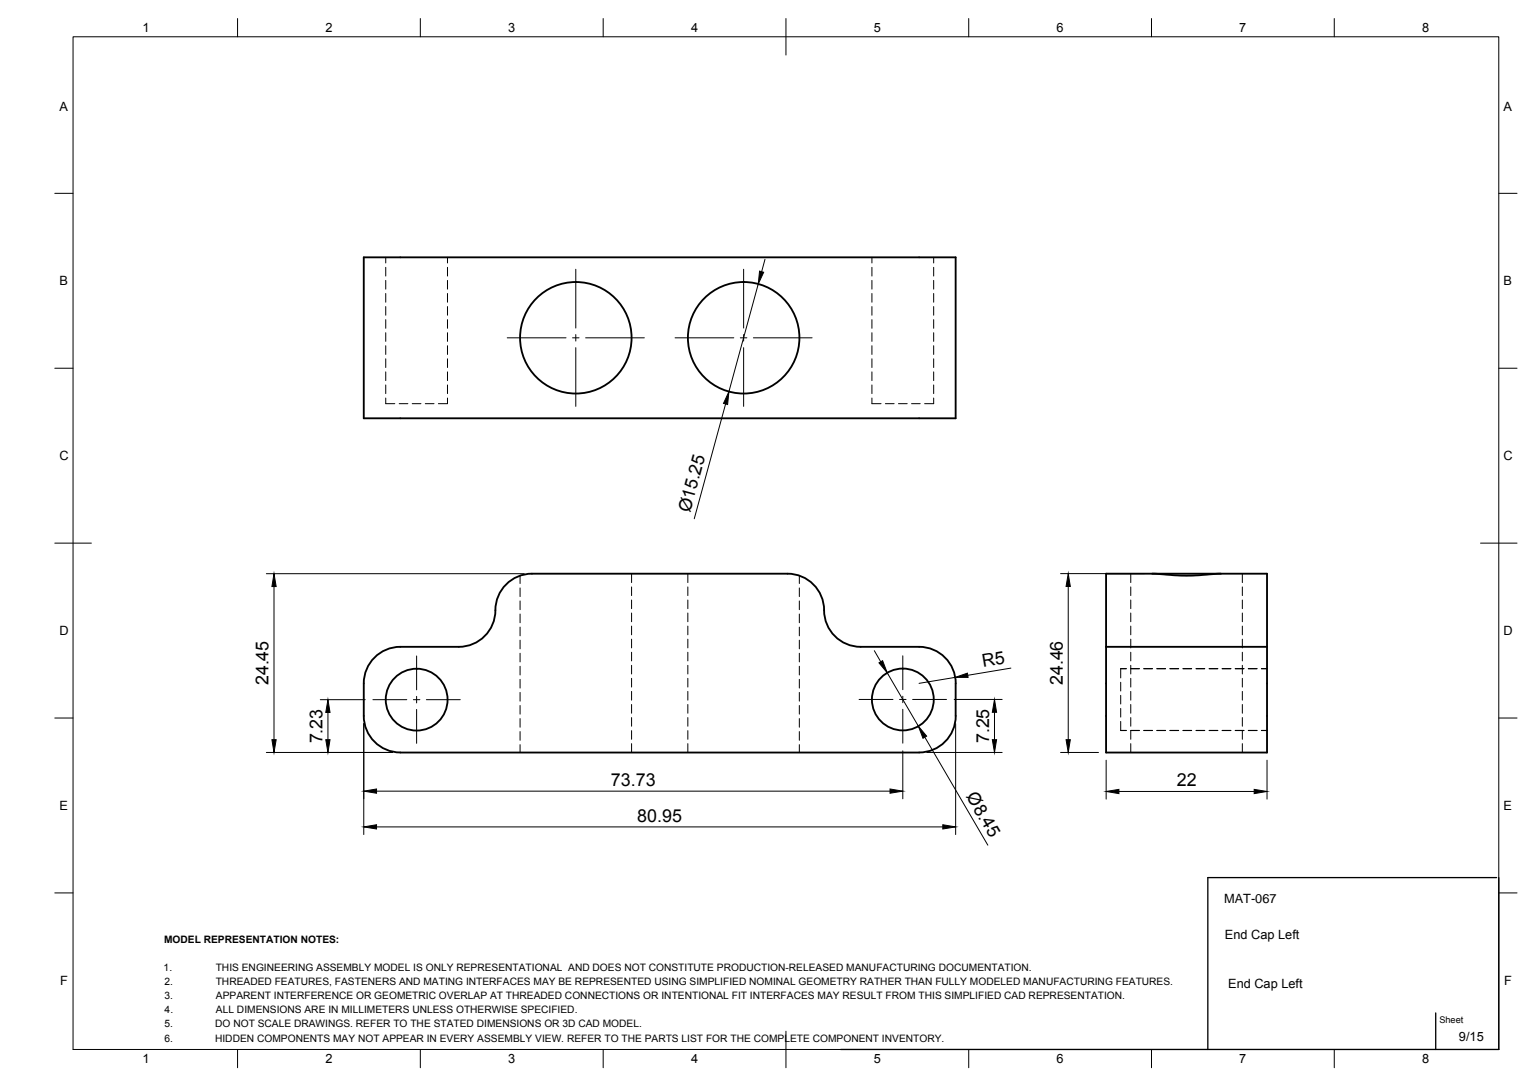
ISO-10303-21;
HEADER;
/* Generated by software containing ST-Developer
 * from STEP Tools, Inc. (www.steptools.com) 
 */

FILE_DESCRIPTION(
/* description */ ('CAx-IF Rec.Pracs.---Representation and Presentation of Product Manufa
cturing Information (PMI)---4.0---2014-10-13'),
/* implementation_level */ '2;1');

FILE_NAME(
/* name */ 'End Cap Left.step',
/* time_stamp */ '2026-10-24T16:02:03-07:00',
/* author */ (''),
/* organization */ (''),
/* preprocessor_version */ 'ST-DEVELOPER v20.2',
/* originating_system */ 'Autodesk Translation Framework v15.17.0.0',
/* authorisation */ '');

FILE_SCHEMA (('AP242_MANAGED_MODEL_BASED_3D_ENGINEERING_MIM_LF { 1 0 10303 442 2 1 4 }'));
ENDSEC;

DATA;
#10=MECHANICAL_DESIGN_GEOMETRIC_PRESENTATION_REPRESENTATION('',(#354),#6348);
#332=SHAPE_REPRESENTATION_RELATIONSHIP('SRR','None',#6483,#343);
#343=ADVANCED_BREP_SHAPE_REPRESENTATION('',(#365),#6331);
#354=STYLED_ITEM('',(#6604),#365);
#365=MANIFOLD_SOLID_BREP('Body1',#3393);
#382=B_SPLINE_CURVE_WITH_KNOTS('',3,(#5983,#5984,#5985,#5986,#5987,#5988),
 .UNSPECIFIED.,.F.,.F.,(4,2,4),(3.46797062946804,3.66737221611079,3.95578831781598),
 .UNSPECIFIED.);
#383=B_SPLINE_CURVE_WITH_KNOTS('',3,(#5989,#5990,#5991,#5992,#5993,#5994),
 .UNSPECIFIED.,.F.,.F.,(4,2,4),(3.95578831781598,4.24420441952117,4.44360600616391),
 .UNSPECIFIED.);
#384=B_SPLINE_CURVE_WITH_KNOTS('',3,(#5997,#5998,#5999,#6000,#6001,#6002,
#6003,#6004,#6005,#6006),.UNSPECIFIED.,.F.,.F.,(4,2,2,2,4),(-4.44360600616391,
-4.24420441952117,-3.95578831781597,-3.66737221611078,-3.46797062946804),
 .UNSPECIFIED.);
#433=CYLINDRICAL_SURFACE('',#3738,0.004225);
#434=CYLINDRICAL_SURFACE('',#3742,0.004225);
#435=CYLINDRICAL_SURFACE('',#3765,0.005);
#436=CYLINDRICAL_SURFACE('',#3766,0.005);
#437=CYLINDRICAL_SURFACE('',#3767,0.005);
#438=CYLINDRICAL_SURFACE('',#3768,0.005);
#439=CYLINDRICAL_SURFACE('',#3773,0.007625);
#440=CYLINDRICAL_SURFACE('',#3774,0.007625);
#441=CYLINDRICAL_SURFACE('',#3775,0.005);
#442=CYLINDRICAL_SURFACE('',#3776,0.005);
#443=CYLINDRICAL_SURFACE('',#3777,0.005);
#444=CYLINDRICAL_SURFACE('',#3778,0.005);
#484=FACE_BOUND('',#986,.T.);
#485=FACE_BOUND('',#987,.T.);
#486=FACE_BOUND('',#993,.T.);
#487=FACE_BOUND('',#994,.T.);
#611=CIRCLE('',#3735,0.007625);
#612=CIRCLE('',#3736,0.007625);
#613=CIRCLE('',#3739,0.004225);
#614=CIRCLE('',#3740,0.004225);
#615=CIRCLE('',#3743,0.004225);
#616=CIRCLE('',#3744,0.004225);
#617=CIRCLE('',#3746,0.005);
#618=CIRCLE('',#3747,0.005);
#619=CIRCLE('',#3748,0.005);
#620=CIRCLE('',#3749,0.005);
#621=CIRCLE('',#3750,0.005);
#622=CIRCLE('',#3751,0.005);
#623=CIRCLE('',#3752,0.005);
#624=CIRCLE('',#3753,0.005);
#625=CIRCLE('',#3757,0.005);
#626=CIRCLE('',#3758,0.005);
#627=CIRCLE('',#3759,0.005);
#628=CIRCLE('',#3760,0.005);
#629=CIRCLE('',#3761,0.005);
#630=CIRCLE('',#3762,0.005);
#631=CIRCLE('',#3763,0.005);
#632=CIRCLE('',#3764,0.005);
#633=CIRCLE('',#3770,0.007625);
#634=CIRCLE('',#3771,0.007625);
#635=CIRCLE('',#3772,0.007625);
#792=FACE_OUTER_BOUND('',#983,.T.);
#793=FACE_OUTER_BOUND('',#984,.T.);
#794=FACE_OUTER_BOUND('',#985,.T.);
#795=FACE_OUTER_BOUND('',#988,.T.);
#796=FACE_OUTER_BOUND('',#989,.T.);
#797=FACE_OUTER_BOUND('',#990,.T.);
#798=FACE_OUTER_BOUND('',#991,.T.);
#799=FACE_OUTER_BOUND('',#992,.T.);
#800=FACE_OUTER_BOUND('',#995,.T.);
#801=FACE_OUTER_BOUND('',#996,.T.);
#802=FACE_OUTER_BOUND('',#997,.T.);
#803=FACE_OUTER_BOUND('',#998,.T.);
#804=FACE_OUTER_BOUND('',#999,.T.);
#805=FACE_OUTER_BOUND('',#1000,.T.);
#806=FACE_OUTER_BOUND('',#1001,.T.);
#807=FACE_OUTER_BOUND('',#1002,.T.);
#808=FACE_OUTER_BOUND('',#1003,.T.);
#809=FACE_OUTER_BOUND('',#1004,.T.);
#810=FACE_OUTER_BOUND('',#1005,.T.);
#811=FACE_OUTER_BOUND('',#1006,.T.);
#812=FACE_OUTER_BOUND('',#1007,.T.);
#813=FACE_OUTER_BOUND('',#1008,.T.);
#983=EDGE_LOOP('',(#2843,#2844,#2845,#2846));
#984=EDGE_LOOP('',(#2847,#2848,#2849,#2850));
#985=EDGE_LOOP('',(#2851,#2852,#2853,#2854));
#986=EDGE_LOOP('',(#2855));
#987=EDGE_LOOP('',(#2856));
#988=EDGE_LOOP('',(#2857,#2858,#2859,#2860));
#989=EDGE_LOOP('',(#2861,#2862,#2863,#2864));
#990=EDGE_LOOP('',(#2865,#2866,#2867,#2868));
#991=EDGE_LOOP('',(#2869,#2870,#2871,#2872));
#992=EDGE_LOOP('',(#2873,#2874,#2875,#2876,#2877,#2878,#2879,#2880,#2881,
#2882,#2883,#2884,#2885,#2886));
#993=EDGE_LOOP('',(#2887));
#994=EDGE_LOOP('',(#2888));
#995=EDGE_LOOP('',(#2889));
#996=EDGE_LOOP('',(#2890));
#997=EDGE_LOOP('',(#2891,#2892,#2893,#2894,#2895,#2896,#2897,#2898,#2899,
#2900,#2901,#2902,#2903,#2904));
#998=EDGE_LOOP('',(#2905,#2906,#2907,#2908));
#999=EDGE_LOOP('',(#2909,#2910,#2911,#2912));
#1000=EDGE_LOOP('',(#2913,#2914,#2915,#2916));
#1001=EDGE_LOOP('',(#2917,#2918,#2919,#2920));
#1002=EDGE_LOOP('',(#2921,#2922,#2923,#2924,#2925,#2926,#2927,#2928,#2929));
#1003=EDGE_LOOP('',(#2930,#2931,#2932,#2933,#2934,#2935));
#1004=EDGE_LOOP('',(#2936,#2937,#2938,#2939,#2940,#2941));
#1005=EDGE_LOOP('',(#2942,#2943,#2944,#2945,#2946,#2947));
#1006=EDGE_LOOP('',(#2948,#2949,#2950,#2951));
#1007=EDGE_LOOP('',(#2952,#2953,#2954,#2955,#2956,#2957,#2958));
#1008=EDGE_LOOP('',(#2959,#2960,#2961,#2962));
#1250=LINE('',#5875,#1483);
#1251=LINE('',#5877,#1484);
#1252=LINE('',#5879,#1485);
#1253=LINE('',#5880,#1486);
#1254=LINE('',#5884,#1487);
#1255=LINE('',#5886,#1488);
#1256=LINE('',#5888,#1489);
#1257=LINE('',#5889,#1490);
#1258=LINE('',#5893,#1491);
#1259=LINE('',#5895,#1492);
#1260=LINE('',#5897,#1493);
#1261=LINE('',#5898,#1494);
#1262=LINE('',#5906,#1495);
#1263=LINE('',#5908,#1496);
#1264=LINE('',#5910,#1497);
#1265=LINE('',#5911,#1498);
#1266=LINE('',#5916,#1499);
#1267=LINE('',#5921,#1500);
#1268=LINE('',#5923,#1501);
#1269=LINE('',#5925,#1502);
#1270=LINE('',#5926,#1503);
#1271=LINE('',#5931,#1504);
#1272=LINE('',#5936,#1505);
#1273=LINE('',#5955,#1506);
#1274=LINE('',#5969,#1507);
#1275=LINE('',#5974,#1508);
#1276=LINE('',#5976,#1509);
#1277=LINE('',#5979,#1510);
#1278=LINE('',#5982,#1511);
#1279=LINE('',#5996,#1512);
#1280=LINE('',#6008,#1513);
#1281=LINE('',#6011,#1514);
#1483=VECTOR('',#4576,1.);
#1484=VECTOR('',#4577,1.);
#1485=VECTOR('',#4578,1.);
#1486=VECTOR('',#4579,1.);
#1487=VECTOR('',#4582,1.);
#1488=VECTOR('',#4583,1.);
#1489=VECTOR('',#4584,1.);
#1490=VECTOR('',#4585,1.);
#1491=VECTOR('',#4588,1.);
#1492=VECTOR('',#4589,1.);
#1493=VECTOR('',#4590,1.);
#1494=VECTOR('',#4591,1.);
#1495=VECTOR('',#4598,1.);
#1496=VECTOR('',#4599,1.);
#1497=VECTOR('',#4600,1.);
#1498=VECTOR('',#4601,1.);
#1499=VECTOR('',#4606,0.004225);
#1500=VECTOR('',#4611,1.);
#1501=VECTOR('',#4612,1.);
#1502=VECTOR('',#4613,1.);
#1503=VECTOR('',#4614,1.);
#1504=VECTOR('',#4619,0.004225);
#1505=VECTOR('',#4624,1.);
#1506=VECTOR('',#4651,1.);
#1507=VECTOR('',#4674,1.);
#1508=VECTOR('',#4679,1.);
#1509=VECTOR('',#4680,1.);
#1510=VECTOR('',#4683,1.);
#1511=VECTOR('',#4686,0.007625);
#1512=VECTOR('',#4689,0.007625);
#1513=VECTOR('',#4692,1.);
#1514=VECTOR('',#4697,1.);
#1736=VERTEX_POINT('',#5873);
#1737=VERTEX_POINT('',#5874);
#1738=VERTEX_POINT('',#5876);
#1739=VERTEX_POINT('',#5878);
#1740=VERTEX_POINT('',#5882);
#1741=VERTEX_POINT('',#5883);
#1742=VERTEX_POINT('',#5885);
#1743=VERTEX_POINT('',#5887);
#1744=VERTEX_POINT('',#5891);
#1745=VERTEX_POINT('',#5892);
#1746=VERTEX_POINT('',#5894);
#1747=VERTEX_POINT('',#5896);
#1748=VERTEX_POINT('',#5899);
#1749=VERTEX_POINT('',#5901);
#1750=VERTEX_POINT('',#5904);
#1751=VERTEX_POINT('',#5905);
#1752=VERTEX_POINT('',#5907);
#1753=VERTEX_POINT('',#5909);
#1754=VERTEX_POINT('',#5913);
#1755=VERTEX_POINT('',#5915);
#1756=VERTEX_POINT('',#5919);
#1757=VERTEX_POINT('',#5920);
#1758=VERTEX_POINT('',#5922);
#1759=VERTEX_POINT('',#5924);
#1760=VERTEX_POINT('',#5928);
#1761=VERTEX_POINT('',#5930);
#1762=VERTEX_POINT('',#5934);
#1763=VERTEX_POINT('',#5935);
#1764=VERTEX_POINT('',#5937);
#1765=VERTEX_POINT('',#5944);
#1766=VERTEX_POINT('',#5950);
#1767=VERTEX_POINT('',#5952);
#1768=VERTEX_POINT('',#5954);
#1769=VERTEX_POINT('',#5956);
#1770=VERTEX_POINT('',#5968);
#1771=VERTEX_POINT('',#5970);
#1772=VERTEX_POINT('',#5972);
#1773=VERTEX_POINT('',#5975);
#1774=VERTEX_POINT('',#5977);
#1775=VERTEX_POINT('',#5981);
#2120=EDGE_CURVE('',#1736,#1737,#1250,.T.);
#2121=EDGE_CURVE('',#1736,#1738,#1251,.F.);
#2122=EDGE_CURVE('',#1738,#1739,#1252,.T.);
#2123=EDGE_CURVE('',#1739,#1737,#1253,.T.);
#2124=EDGE_CURVE('',#1740,#1741,#1254,.T.);
#2125=EDGE_CURVE('',#1741,#1742,#1255,.T.);
#2126=EDGE_CURVE('',#1743,#1742,#1256,.T.);
#2127=EDGE_CURVE('',#1743,#1740,#1257,.F.);
#2128=EDGE_CURVE('',#1744,#1745,#1258,.T.);
#2129=EDGE_CURVE('',#1744,#1746,#1259,.T.);
#2130=EDGE_CURVE('',#1746,#1747,#1260,.T.);
#2131=EDGE_CURVE('',#1747,#1745,#1261,.F.);
#2132=EDGE_CURVE('',#1748,#1748,#611,.T.);
#2133=EDGE_CURVE('',#1749,#1749,#612,.T.);
#2134=EDGE_CURVE('',#1750,#1751,#1262,.T.);
#2135=EDGE_CURVE('',#1750,#1752,#1263,.T.);
#2136=EDGE_CURVE('',#1752,#1753,#1264,.T.);
#2137=EDGE_CURVE('',#1753,#1751,#1265,.F.);
#2138=EDGE_CURVE('',#1754,#1754,#613,.T.);
#2139=EDGE_CURVE('',#1754,#1755,#1266,.T.);
#2140=EDGE_CURVE('',#1755,#1755,#614,.T.);
#2141=EDGE_CURVE('',#1756,#1757,#1267,.T.);
#2142=EDGE_CURVE('',#1757,#1758,#1268,.T.);
#2143=EDGE_CURVE('',#1759,#1758,#1269,.T.);
#2144=EDGE_CURVE('',#1759,#1756,#1270,.F.);
#2145=EDGE_CURVE('',#1760,#1760,#615,.T.);
#2146=EDGE_CURVE('',#1760,#1761,#1271,.T.);
#2147=EDGE_CURVE('',#1761,#1761,#616,.T.);
#2148=EDGE_CURVE('',#1762,#1763,#1272,.T.);
#2149=EDGE_CURVE('',#1763,#1764,#617,.F.);
#2150=EDGE_CURVE('',#1764,#1736,#618,.T.);
#2151=EDGE_CURVE('',#1737,#1753,#619,.F.);
#2152=EDGE_CURVE('',#1752,#1747,#620,.F.);
#2153=EDGE_CURVE('',#1746,#1743,#621,.F.);
#2154=EDGE_CURVE('',#1742,#1759,#622,.F.);
#2155=EDGE_CURVE('',#1758,#1765,#623,.T.);
#2156=EDGE_CURVE('',#1765,#1762,#624,.F.);
#2157=EDGE_CURVE('',#1738,#1766,#625,.F.);
#2158=EDGE_CURVE('',#1766,#1767,#626,.T.);
#2159=EDGE_CURVE('',#1768,#1767,#1273,.T.);
#2160=EDGE_CURVE('',#1768,#1769,#627,.T.);
#2161=EDGE_CURVE('',#1769,#1757,#628,.F.);
#2162=EDGE_CURVE('',#1756,#1741,#629,.T.);
#2163=EDGE_CURVE('',#1740,#1744,#630,.T.);
#2164=EDGE_CURVE('',#1745,#1750,#631,.T.);
#2165=EDGE_CURVE('',#1751,#1739,#632,.T.);
#2166=EDGE_CURVE('',#1767,#1770,#1274,.T.);
#2167=EDGE_CURVE('',#1771,#1770,#633,.T.);
#2168=EDGE_CURVE('',#1772,#1771,#634,.T.);
#2169=EDGE_CURVE('',#1772,#1763,#1275,.T.);
#2170=EDGE_CURVE('',#1762,#1773,#1276,.F.);
#2171=EDGE_CURVE('',#1774,#1773,#635,.T.);
#2172=EDGE_CURVE('',#1774,#1768,#1277,.F.);
#2173=EDGE_CURVE('',#1749,#1775,#1278,.T.);
#2174=EDGE_CURVE('',#1775,#1774,#382,.F.);
#2175=EDGE_CURVE('',#1773,#1775,#383,.F.);
#2176=EDGE_CURVE('',#1748,#1771,#1279,.T.);
#2177=EDGE_CURVE('',#1770,#1772,#384,.T.);
#2178=EDGE_CURVE('',#1764,#1766,#1280,.F.);
#2179=EDGE_CURVE('',#1769,#1765,#1281,.T.);
#2843=ORIENTED_EDGE('',*,*,#2120,.F.);
#2844=ORIENTED_EDGE('',*,*,#2121,.T.);
#2845=ORIENTED_EDGE('',*,*,#2122,.T.);
#2846=ORIENTED_EDGE('',*,*,#2123,.T.);
#2847=ORIENTED_EDGE('',*,*,#2124,.T.);
#2848=ORIENTED_EDGE('',*,*,#2125,.T.);
#2849=ORIENTED_EDGE('',*,*,#2126,.F.);
#2850=ORIENTED_EDGE('',*,*,#2127,.T.);
#2851=ORIENTED_EDGE('',*,*,#2128,.F.);
#2852=ORIENTED_EDGE('',*,*,#2129,.T.);
#2853=ORIENTED_EDGE('',*,*,#2130,.T.);
#2854=ORIENTED_EDGE('',*,*,#2131,.T.);
#2855=ORIENTED_EDGE('',*,*,#2132,.T.);
#2856=ORIENTED_EDGE('',*,*,#2133,.T.);
#2857=ORIENTED_EDGE('',*,*,#2134,.F.);
#2858=ORIENTED_EDGE('',*,*,#2135,.T.);
#2859=ORIENTED_EDGE('',*,*,#2136,.T.);
#2860=ORIENTED_EDGE('',*,*,#2137,.T.);
#2861=ORIENTED_EDGE('',*,*,#2138,.T.);
#2862=ORIENTED_EDGE('',*,*,#2139,.T.);
#2863=ORIENTED_EDGE('',*,*,#2140,.F.);
#2864=ORIENTED_EDGE('',*,*,#2139,.F.);
#2865=ORIENTED_EDGE('',*,*,#2141,.T.);
#2866=ORIENTED_EDGE('',*,*,#2142,.T.);
#2867=ORIENTED_EDGE('',*,*,#2143,.F.);
#2868=ORIENTED_EDGE('',*,*,#2144,.T.);
#2869=ORIENTED_EDGE('',*,*,#2145,.T.);
#2870=ORIENTED_EDGE('',*,*,#2146,.T.);
#2871=ORIENTED_EDGE('',*,*,#2147,.F.);
#2872=ORIENTED_EDGE('',*,*,#2146,.F.);
#2873=ORIENTED_EDGE('',*,*,#2148,.T.);
#2874=ORIENTED_EDGE('',*,*,#2149,.T.);
#2875=ORIENTED_EDGE('',*,*,#2150,.T.);
#2876=ORIENTED_EDGE('',*,*,#2120,.T.);
#2877=ORIENTED_EDGE('',*,*,#2151,.T.);
#2878=ORIENTED_EDGE('',*,*,#2136,.F.);
#2879=ORIENTED_EDGE('',*,*,#2152,.T.);
#2880=ORIENTED_EDGE('',*,*,#2130,.F.);
#2881=ORIENTED_EDGE('',*,*,#2153,.T.);
#2882=ORIENTED_EDGE('',*,*,#2126,.T.);
#2883=ORIENTED_EDGE('',*,*,#2154,.T.);
#2884=ORIENTED_EDGE('',*,*,#2143,.T.);
#2885=ORIENTED_EDGE('',*,*,#2155,.T.);
#2886=ORIENTED_EDGE('',*,*,#2156,.T.);
#2887=ORIENTED_EDGE('',*,*,#2140,.T.);
#2888=ORIENTED_EDGE('',*,*,#2147,.T.);
#2889=ORIENTED_EDGE('',*,*,#2145,.F.);
#2890=ORIENTED_EDGE('',*,*,#2138,.F.);
#2891=ORIENTED_EDGE('',*,*,#2122,.F.);
#2892=ORIENTED_EDGE('',*,*,#2157,.T.);
#2893=ORIENTED_EDGE('',*,*,#2158,.T.);
#2894=ORIENTED_EDGE('',*,*,#2159,.F.);
#2895=ORIENTED_EDGE('',*,*,#2160,.T.);
#2896=ORIENTED_EDGE('',*,*,#2161,.T.);
#2897=ORIENTED_EDGE('',*,*,#2141,.F.);
#2898=ORIENTED_EDGE('',*,*,#2162,.T.);
#2899=ORIENTED_EDGE('',*,*,#2124,.F.);
#2900=ORIENTED_EDGE('',*,*,#2163,.T.);
#2901=ORIENTED_EDGE('',*,*,#2128,.T.);
#2902=ORIENTED_EDGE('',*,*,#2164,.T.);
#2903=ORIENTED_EDGE('',*,*,#2134,.T.);
#2904=ORIENTED_EDGE('',*,*,#2165,.T.);
#2905=ORIENTED_EDGE('',*,*,#2162,.F.);
#2906=ORIENTED_EDGE('',*,*,#2144,.F.);
#2907=ORIENTED_EDGE('',*,*,#2154,.F.);
#2908=ORIENTED_EDGE('',*,*,#2125,.F.);
#2909=ORIENTED_EDGE('',*,*,#2163,.F.);
#2910=ORIENTED_EDGE('',*,*,#2127,.F.);
#2911=ORIENTED_EDGE('',*,*,#2153,.F.);
#2912=ORIENTED_EDGE('',*,*,#2129,.F.);
#2913=ORIENTED_EDGE('',*,*,#2164,.F.);
#2914=ORIENTED_EDGE('',*,*,#2131,.F.);
#2915=ORIENTED_EDGE('',*,*,#2152,.F.);
#2916=ORIENTED_EDGE('',*,*,#2135,.F.);
#2917=ORIENTED_EDGE('',*,*,#2165,.F.);
#2918=ORIENTED_EDGE('',*,*,#2137,.F.);
#2919=ORIENTED_EDGE('',*,*,#2151,.F.);
#2920=ORIENTED_EDGE('',*,*,#2123,.F.);
#2921=ORIENTED_EDGE('',*,*,#2159,.T.);
#2922=ORIENTED_EDGE('',*,*,#2166,.T.);
#2923=ORIENTED_EDGE('',*,*,#2167,.F.);
#2924=ORIENTED_EDGE('',*,*,#2168,.F.);
#2925=ORIENTED_EDGE('',*,*,#2169,.T.);
#2926=ORIENTED_EDGE('',*,*,#2148,.F.);
#2927=ORIENTED_EDGE('',*,*,#2170,.T.);
#2928=ORIENTED_EDGE('',*,*,#2171,.F.);
#2929=ORIENTED_EDGE('',*,*,#2172,.T.);
#2930=ORIENTED_EDGE('',*,*,#2133,.F.);
#2931=ORIENTED_EDGE('',*,*,#2173,.T.);
#2932=ORIENTED_EDGE('',*,*,#2174,.T.);
#2933=ORIENTED_EDGE('',*,*,#2171,.T.);
#2934=ORIENTED_EDGE('',*,*,#2175,.T.);
#2935=ORIENTED_EDGE('',*,*,#2173,.F.);
#2936=ORIENTED_EDGE('',*,*,#2132,.F.);
#2937=ORIENTED_EDGE('',*,*,#2176,.T.);
#2938=ORIENTED_EDGE('',*,*,#2167,.T.);
#2939=ORIENTED_EDGE('',*,*,#2177,.T.);
#2940=ORIENTED_EDGE('',*,*,#2168,.T.);
#2941=ORIENTED_EDGE('',*,*,#2176,.F.);
#2942=ORIENTED_EDGE('',*,*,#2166,.F.);
#2943=ORIENTED_EDGE('',*,*,#2158,.F.);
#2944=ORIENTED_EDGE('',*,*,#2178,.F.);
#2945=ORIENTED_EDGE('',*,*,#2149,.F.);
#2946=ORIENTED_EDGE('',*,*,#2169,.F.);
#2947=ORIENTED_EDGE('',*,*,#2177,.F.);
#2948=ORIENTED_EDGE('',*,*,#2157,.F.);
#2949=ORIENTED_EDGE('',*,*,#2121,.F.);
#2950=ORIENTED_EDGE('',*,*,#2150,.F.);
#2951=ORIENTED_EDGE('',*,*,#2178,.T.);
#2952=ORIENTED_EDGE('',*,*,#2179,.F.);
#2953=ORIENTED_EDGE('',*,*,#2160,.F.);
#2954=ORIENTED_EDGE('',*,*,#2172,.F.);
#2955=ORIENTED_EDGE('',*,*,#2174,.F.);
#2956=ORIENTED_EDGE('',*,*,#2175,.F.);
#2957=ORIENTED_EDGE('',*,*,#2170,.F.);
#2958=ORIENTED_EDGE('',*,*,#2156,.F.);
#2959=ORIENTED_EDGE('',*,*,#2161,.F.);
#2960=ORIENTED_EDGE('',*,*,#2179,.T.);
#2961=ORIENTED_EDGE('',*,*,#2155,.F.);
#2962=ORIENTED_EDGE('',*,*,#2142,.F.);
#3187=PLANE('',#3732);
#3188=PLANE('',#3733);
#3189=PLANE('',#3734);
#3190=PLANE('',#3737);
#3191=PLANE('',#3741);
#3192=PLANE('',#3745);
#3193=PLANE('',#3754);
#3194=PLANE('',#3755);
#3195=PLANE('',#3756);
#3196=PLANE('',#3769);
#3315=ADVANCED_FACE('',(#792),#3187,.T.);
#3316=ADVANCED_FACE('',(#793),#3188,.T.);
#3317=ADVANCED_FACE('',(#794,#484,#485),#3189,.F.);
#3318=ADVANCED_FACE('',(#795),#3190,.F.);
#3319=ADVANCED_FACE('',(#796),#433,.F.);
#3320=ADVANCED_FACE('',(#797),#3191,.T.);
#3321=ADVANCED_FACE('',(#798),#434,.F.);
#3322=ADVANCED_FACE('',(#799,#486,#487),#3192,.F.);
#3323=ADVANCED_FACE('',(#800),#3193,.F.);
#3324=ADVANCED_FACE('',(#801),#3194,.F.);
#3325=ADVANCED_FACE('',(#802),#3195,.T.);
#3326=ADVANCED_FACE('',(#803),#435,.T.);
#3327=ADVANCED_FACE('',(#804),#436,.T.);
#3328=ADVANCED_FACE('',(#805),#437,.T.);
#3329=ADVANCED_FACE('',(#806),#438,.T.);
#3330=ADVANCED_FACE('',(#807),#3196,.T.);
#3331=ADVANCED_FACE('',(#808),#439,.F.);
#3332=ADVANCED_FACE('',(#809),#440,.F.);
#3333=ADVANCED_FACE('',(#810),#441,.T.);
#3334=ADVANCED_FACE('',(#811),#442,.F.);
#3335=ADVANCED_FACE('',(#812),#443,.T.);
#3336=ADVANCED_FACE('',(#813),#444,.F.);
#3393=CLOSED_SHELL('',(#3315,#3316,#3317,#3318,#3319,#3320,#3321,#3322,
#3323,#3324,#3325,#3326,#3327,#3328,#3329,#3330,#3331,#3332,#3333,#3334,
#3335,#3336));
#3731=AXIS2_PLACEMENT_3D('',#5871,#4572,#4573);
#3732=AXIS2_PLACEMENT_3D('',#5872,#4574,#4575);
#3733=AXIS2_PLACEMENT_3D('',#5881,#4580,#4581);
#3734=AXIS2_PLACEMENT_3D('',#5890,#4586,#4587);
#3735=AXIS2_PLACEMENT_3D('',#5900,#4592,#4593);
#3736=AXIS2_PLACEMENT_3D('',#5902,#4594,#4595);
#3737=AXIS2_PLACEMENT_3D('',#5903,#4596,#4597);
#3738=AXIS2_PLACEMENT_3D('',#5912,#4602,#4603);
#3739=AXIS2_PLACEMENT_3D('',#5914,#4604,#4605);
#3740=AXIS2_PLACEMENT_3D('',#5917,#4607,#4608);
#3741=AXIS2_PLACEMENT_3D('',#5918,#4609,#4610);
#3742=AXIS2_PLACEMENT_3D('',#5927,#4615,#4616);
#3743=AXIS2_PLACEMENT_3D('',#5929,#4617,#4618);
#3744=AXIS2_PLACEMENT_3D('',#5932,#4620,#4621);
#3745=AXIS2_PLACEMENT_3D('',#5933,#4622,#4623);
#3746=AXIS2_PLACEMENT_3D('',#5938,#4625,#4626);
#3747=AXIS2_PLACEMENT_3D('',#5939,#4627,#4628);
#3748=AXIS2_PLACEMENT_3D('',#5940,#4629,#4630);
#3749=AXIS2_PLACEMENT_3D('',#5941,#4631,#4632);
#3750=AXIS2_PLACEMENT_3D('',#5942,#4633,#4634);
#3751=AXIS2_PLACEMENT_3D('',#5943,#4635,#4636);
#3752=AXIS2_PLACEMENT_3D('',#5945,#4637,#4638);
#3753=AXIS2_PLACEMENT_3D('',#5946,#4639,#4640);
#3754=AXIS2_PLACEMENT_3D('',#5947,#4641,#4642);
#3755=AXIS2_PLACEMENT_3D('',#5948,#4643,#4644);
#3756=AXIS2_PLACEMENT_3D('',#5949,#4645,#4646);
#3757=AXIS2_PLACEMENT_3D('',#5951,#4647,#4648);
#3758=AXIS2_PLACEMENT_3D('',#5953,#4649,#4650);
#3759=AXIS2_PLACEMENT_3D('',#5957,#4652,#4653);
#3760=AXIS2_PLACEMENT_3D('',#5958,#4654,#4655);
#3761=AXIS2_PLACEMENT_3D('',#5959,#4656,#4657);
#3762=AXIS2_PLACEMENT_3D('',#5960,#4658,#4659);
#3763=AXIS2_PLACEMENT_3D('',#5961,#4660,#4661);
#3764=AXIS2_PLACEMENT_3D('',#5962,#4662,#4663);
#3765=AXIS2_PLACEMENT_3D('',#5963,#4664,#4665);
#3766=AXIS2_PLACEMENT_3D('',#5964,#4666,#4667);
#3767=AXIS2_PLACEMENT_3D('',#5965,#4668,#4669);
#3768=AXIS2_PLACEMENT_3D('',#5966,#4670,#4671);
#3769=AXIS2_PLACEMENT_3D('',#5967,#4672,#4673);
#3770=AXIS2_PLACEMENT_3D('',#5971,#4675,#4676);
#3771=AXIS2_PLACEMENT_3D('',#5973,#4677,#4678);
#3772=AXIS2_PLACEMENT_3D('',#5978,#4681,#4682);
#3773=AXIS2_PLACEMENT_3D('',#5980,#4684,#4685);
#3774=AXIS2_PLACEMENT_3D('',#5995,#4687,#4688);
#3775=AXIS2_PLACEMENT_3D('',#6007,#4690,#4691);
#3776=AXIS2_PLACEMENT_3D('',#6009,#4693,#4694);
#3777=AXIS2_PLACEMENT_3D('',#6010,#4695,#4696);
#3778=AXIS2_PLACEMENT_3D('',#6012,#4698,#4699);
#4572=DIRECTION('axis',(0.,0.,1.));
#4573=DIRECTION('refdir',(1.,0.,0.));
#4574=DIRECTION('center_axis',(0.,-1.,8.57182693503055E-17));
#4575=DIRECTION('ref_axis',(0.,-8.57182693503055E-17,-1.));
#4576=DIRECTION('',(0.,-8.57182693503055E-17,-1.));
#4577=DIRECTION('',(1.,0.,0.));
#4578=DIRECTION('',(0.,-8.57182693503055E-17,-1.));
#4579=DIRECTION('',(1.,0.,0.));
#4580=DIRECTION('center_axis',(0.,0.,1.));
#4581=DIRECTION('ref_axis',(1.,0.,0.));
#4582=DIRECTION('',(0.,-1.,0.));
#4583=DIRECTION('',(1.,0.,0.));
#4584=DIRECTION('',(0.,-1.,0.));
#4585=DIRECTION('',(1.,0.,0.));
#4586=DIRECTION('center_axis',(0.,-1.,6.42887020127291E-17));
#4587=DIRECTION('ref_axis',(0.,-6.42887020127291E-17,-1.));
#4588=DIRECTION('',(0.,-6.42887020127291E-17,-1.));
#4589=DIRECTION('',(1.,0.,0.));
#4590=DIRECTION('',(0.,-6.42887020127291E-17,-1.));
#4591=DIRECTION('',(1.,0.,0.));
#4592=DIRECTION('center_axis',(0.,-1.,6.42887020127291E-17));
#4593=DIRECTION('ref_axis',(0.,-6.42887020127291E-17,-1.));
#4594=DIRECTION('center_axis',(0.,-1.,6.42887020127291E-17));
#4595=DIRECTION('ref_axis',(0.,-6.42887020127291E-17,-1.));
#4596=DIRECTION('center_axis',(0.,0.,1.));
#4597=DIRECTION('ref_axis',(1.,0.,0.));
#4598=DIRECTION('',(0.,-1.,0.));
#4599=DIRECTION('',(1.,0.,0.));
#4600=DIRECTION('',(0.,-1.,0.));
#4601=DIRECTION('',(1.,0.,0.));
#4602=DIRECTION('center_axis',(1.,0.,0.));
#4603=DIRECTION('ref_axis',(0.,0.,-1.));
#4604=DIRECTION('center_axis',(-1.,0.,0.));
#4605=DIRECTION('ref_axis',(0.,0.,1.));
#4606=DIRECTION('',(1.,0.,0.));
#4607=DIRECTION('center_axis',(-1.,0.,0.));
#4608=DIRECTION('ref_axis',(0.,0.,1.));
#4609=DIRECTION('center_axis',(0.,-1.,8.57182693503055E-17));
#4610=DIRECTION('ref_axis',(0.,-8.57182693503055E-17,-1.));
#4611=DIRECTION('',(0.,-8.57182693503055E-17,-1.));
#4612=DIRECTION('',(1.,0.,0.));
#4613=DIRECTION('',(0.,-8.57182693503055E-17,-1.));
#4614=DIRECTION('',(1.,0.,0.));
#4615=DIRECTION('center_axis',(1.,0.,0.));
#4616=DIRECTION('ref_axis',(0.,0.,-1.));
#4617=DIRECTION('center_axis',(-1.,0.,0.));
#4618=DIRECTION('ref_axis',(0.,0.,1.));
#4619=DIRECTION('',(1.,0.,0.));
#4620=DIRECTION('center_axis',(-1.,0.,0.));
#4621=DIRECTION('ref_axis',(0.,0.,1.));
#4622=DIRECTION('center_axis',(-1.,0.,0.));
#4623=DIRECTION('ref_axis',(0.,-1.,0.));
#4624=DIRECTION('',(0.,-8.57182693503055E-17,-1.));
#4625=DIRECTION('center_axis',(-1.,0.,0.));
#4626=DIRECTION('ref_axis',(0.,0.,1.));
#4627=DIRECTION('center_axis',(-1.,0.,0.));
#4628=DIRECTION('ref_axis',(0.,0.,1.));
#4629=DIRECTION('center_axis',(-1.,0.,0.));
#4630=DIRECTION('ref_axis',(0.,0.,1.));
#4631=DIRECTION('center_axis',(-1.,0.,0.));
#4632=DIRECTION('ref_axis',(0.,0.,1.));
#4633=DIRECTION('center_axis',(-1.,0.,0.));
#4634=DIRECTION('ref_axis',(0.,0.,1.));
#4635=DIRECTION('center_axis',(-1.,0.,0.));
#4636=DIRECTION('ref_axis',(0.,0.,1.));
#4637=DIRECTION('center_axis',(-1.,0.,0.));
#4638=DIRECTION('ref_axis',(0.,0.,1.));
#4639=DIRECTION('center_axis',(-1.,0.,0.));
#4640=DIRECTION('ref_axis',(0.,0.,1.));
#4641=DIRECTION('center_axis',(-1.,0.,0.));
#4642=DIRECTION('ref_axis',(0.,-1.,0.));
#4643=DIRECTION('center_axis',(-1.,0.,0.));
#4644=DIRECTION('ref_axis',(0.,-1.,0.));
#4645=DIRECTION('center_axis',(-1.,0.,0.));
#4646=DIRECTION('ref_axis',(0.,-1.,0.));
#4647=DIRECTION('center_axis',(-1.,0.,0.));
#4648=DIRECTION('ref_axis',(0.,0.,1.));
#4649=DIRECTION('center_axis',(-1.,0.,0.));
#4650=DIRECTION('ref_axis',(0.,0.,1.));
#4651=DIRECTION('',(0.,-8.57182693503055E-17,-1.));
#4652=DIRECTION('center_axis',(-1.,0.,0.));
#4653=DIRECTION('ref_axis',(0.,0.,1.));
#4654=DIRECTION('center_axis',(-1.,0.,0.));
#4655=DIRECTION('ref_axis',(0.,0.,1.));
#4656=DIRECTION('center_axis',(-1.,0.,0.));
#4657=DIRECTION('ref_axis',(0.,0.,1.));
#4658=DIRECTION('center_axis',(-1.,0.,0.));
#4659=DIRECTION('ref_axis',(0.,0.,1.));
#4660=DIRECTION('center_axis',(-1.,0.,0.));
#4661=DIRECTION('ref_axis',(0.,0.,1.));
#4662=DIRECTION('center_axis',(-1.,0.,0.));
#4663=DIRECTION('ref_axis',(0.,0.,1.));
#4664=DIRECTION('center_axis',(1.,0.,0.));
#4665=DIRECTION('ref_axis',(0.,0.,-1.));
#4666=DIRECTION('center_axis',(-1.,0.,0.));
#4667=DIRECTION('ref_axis',(0.,0.,1.));
#4668=DIRECTION('center_axis',(1.,0.,0.));
#4669=DIRECTION('ref_axis',(0.,0.,-1.));
#4670=DIRECTION('center_axis',(-1.,0.,0.));
#4671=DIRECTION('ref_axis',(0.,0.,1.));
#4672=DIRECTION('center_axis',(0.,-1.,8.57182693503055E-17));
#4673=DIRECTION('ref_axis',(1.,0.,0.));
#4674=DIRECTION('',(1.,0.,0.));
#4675=DIRECTION('center_axis',(0.,-1.,8.57182693503055E-17));
#4676=DIRECTION('ref_axis',(0.,-8.57182693503055E-17,-1.));
#4677=DIRECTION('center_axis',(0.,-1.,8.57182693503055E-17));
#4678=DIRECTION('ref_axis',(0.,-8.57182693503055E-17,-1.));
#4679=DIRECTION('',(1.,0.,0.));
#4680=DIRECTION('',(1.,0.,0.));
#4681=DIRECTION('center_axis',(0.,-1.,8.57182693503055E-17));
#4682=DIRECTION('ref_axis',(0.,-8.57182693503055E-17,-1.));
#4683=DIRECTION('',(1.,0.,0.));
#4684=DIRECTION('center_axis',(0.,-1.,8.57182693503055E-17));
#4685=DIRECTION('ref_axis',(0.,-8.57182693503055E-17,-1.));
#4686=DIRECTION('',(0.,-1.,8.57182693503055E-17));
#4687=DIRECTION('center_axis',(0.,-1.,8.57182693503055E-17));
#4688=DIRECTION('ref_axis',(0.,-8.57182693503055E-17,-1.));
#4689=DIRECTION('',(0.,-1.,8.57182693503055E-17));
#4690=DIRECTION('center_axis',(-1.,0.,0.));
#4691=DIRECTION('ref_axis',(0.,0.,1.));
#4692=DIRECTION('',(1.,0.,0.));
#4693=DIRECTION('center_axis',(1.,0.,0.));
#4694=DIRECTION('ref_axis',(0.,0.,-1.));
#4695=DIRECTION('center_axis',(1.,0.,0.));
#4696=DIRECTION('ref_axis',(0.,0.,-1.));
#4697=DIRECTION('',(1.,0.,0.));
#4698=DIRECTION('center_axis',(-1.,0.,0.));
#4699=DIRECTION('ref_axis',(0.,0.,1.));
#5871=CARTESIAN_POINT('',(0.,0.,0.));
#5872=CARTESIAN_POINT('Origin',(-0.06655,-0.0172,0.02565));
#5873=CARTESIAN_POINT('',(-0.04655,-0.0172,-0.001825));
#5874=CARTESIAN_POINT('',(-0.04655,-0.0172,-0.009825));
#5875=CARTESIAN_POINT('',(-0.04655,-0.0172,0.02565));
#5876=CARTESIAN_POINT('',(-0.06855,-0.0172,-0.001825));
#5877=CARTESIAN_POINT('',(-0.06655,-0.0172,-0.001825));
#5878=CARTESIAN_POINT('',(-0.06855,-0.0172,-0.009825));
#5879=CARTESIAN_POINT('',(-0.06855,-0.0172,0.02565));
#5880=CARTESIAN_POINT('',(-0.04655,-0.0172,-0.009825));
#5881=CARTESIAN_POINT('Origin',(-0.06655,-0.009975,0.066125));
#5882=CARTESIAN_POINT('',(-0.06855,-0.00775,0.066125));
#5883=CARTESIAN_POINT('',(-0.06855,-0.0122,0.066125));
#5884=CARTESIAN_POINT('',(-0.06855,-0.009975,0.066125));
#5885=CARTESIAN_POINT('',(-0.04655,-0.0122,0.066125));
#5886=CARTESIAN_POINT('',(-0.06655,-0.0122,0.066125));
#5887=CARTESIAN_POINT('',(-0.04655,-0.00775,0.066125));
#5888=CARTESIAN_POINT('',(-0.04655,-0.009975,0.066125));
#5889=CARTESIAN_POINT('',(-0.06855,-0.00775,0.066125));
#5890=CARTESIAN_POINT('Origin',(-0.06655,-0.00275,0.02565));
#5891=CARTESIAN_POINT('',(-0.06855,-0.00275,0.061125));
#5892=CARTESIAN_POINT('',(-0.06855,-0.00275,-0.009825));
#5893=CARTESIAN_POINT('',(-0.06855,-0.00275,0.02565));
#5894=CARTESIAN_POINT('',(-0.04655,-0.00275,0.061125));
#5895=CARTESIAN_POINT('',(-0.04655,-0.00275,0.061125));
#5896=CARTESIAN_POINT('',(-0.04655,-0.00275,-0.009825));
#5897=CARTESIAN_POINT('',(-0.04655,-0.00275,0.02565));
#5898=CARTESIAN_POINT('',(-0.06655,-0.00275,-0.009825));
#5899=CARTESIAN_POINT('',(-0.05755,-0.00275,0.0218));
#5900=CARTESIAN_POINT('Origin',(-0.05755,-0.00275,0.014175));
#5901=CARTESIAN_POINT('',(-0.05755,-0.00275,0.04475));
#5902=CARTESIAN_POINT('Origin',(-0.05755,-0.00275,0.037125));
#5903=CARTESIAN_POINT('Origin',(-0.06655,-0.009975,-0.014825));
#5904=CARTESIAN_POINT('',(-0.06855,-0.00775,-0.014825));
#5905=CARTESIAN_POINT('',(-0.06855,-0.0122,-0.014825));
#5906=CARTESIAN_POINT('',(-0.06855,-0.009975,-0.014825));
#5907=CARTESIAN_POINT('',(-0.04655,-0.00775,-0.014825));
#5908=CARTESIAN_POINT('',(-0.06655,-0.00775,-0.014825));
#5909=CARTESIAN_POINT('',(-0.04655,-0.0122,-0.014825));
#5910=CARTESIAN_POINT('',(-0.04655,-0.009975,-0.014825));
#5911=CARTESIAN_POINT('',(-0.06855,-0.0122,-0.014825));
#5912=CARTESIAN_POINT('Origin',(-0.06655,-0.009975,-0.0076));
#5913=CARTESIAN_POINT('',(-0.06655,-0.009975,-0.003375));
#5914=CARTESIAN_POINT('Origin',(-0.06655,-0.009975,-0.0076));
#5915=CARTESIAN_POINT('',(-0.04655,-0.009975,-0.003375));
#5916=CARTESIAN_POINT('',(-0.06655,-0.009975,-0.003375));
#5917=CARTESIAN_POINT('Origin',(-0.04655,-0.009975,-0.0076));
#5918=CARTESIAN_POINT('Origin',(-0.06655,-0.0172,0.02565));
#5919=CARTESIAN_POINT('',(-0.06855,-0.0172,0.061125));
#5920=CARTESIAN_POINT('',(-0.06855,-0.0172,0.053125));
#5921=CARTESIAN_POINT('',(-0.06855,-0.0172,0.02565));
#5922=CARTESIAN_POINT('',(-0.04655,-0.0172,0.053125));
#5923=CARTESIAN_POINT('',(-0.04655,-0.0172,0.053125));
#5924=CARTESIAN_POINT('',(-0.04655,-0.0172,0.061125));
#5925=CARTESIAN_POINT('',(-0.04655,-0.0172,0.02565));
#5926=CARTESIAN_POINT('',(-0.06655,-0.0172,0.061125));
#5927=CARTESIAN_POINT('Origin',(-0.06655,-0.01,0.0589));
#5928=CARTESIAN_POINT('',(-0.06655,-0.01,0.063125));
#5929=CARTESIAN_POINT('Origin',(-0.06655,-0.01,0.0589));
#5930=CARTESIAN_POINT('',(-0.04655,-0.01,0.063125));
#5931=CARTESIAN_POINT('',(-0.06655,-0.01,0.063125));
#5932=CARTESIAN_POINT('Origin',(-0.04655,-0.01,0.0589));
#5933=CARTESIAN_POINT('Origin',(-0.04655,0.,0.02565));
#5934=CARTESIAN_POINT('',(-0.04655,-0.0272,0.043125));
#5935=CARTESIAN_POINT('',(-0.04655,-0.0272,0.008175));
#5936=CARTESIAN_POINT('',(-0.04655,-0.0272,0.02565));
#5937=CARTESIAN_POINT('',(-0.04655,-0.0222,0.003175));
#5938=CARTESIAN_POINT('Origin',(-0.04655,-0.0222,0.008175));
#5939=CARTESIAN_POINT('Origin',(-0.04655,-0.0222,-0.001825));
#5940=CARTESIAN_POINT('Origin',(-0.04655,-0.0122,-0.009825));
#5941=CARTESIAN_POINT('Origin',(-0.04655,-0.00775,-0.009825));
#5942=CARTESIAN_POINT('Origin',(-0.04655,-0.00775,0.061125));
#5943=CARTESIAN_POINT('Origin',(-0.04655,-0.0122,0.061125));
#5944=CARTESIAN_POINT('',(-0.04655,-0.0222,0.048125));
#5945=CARTESIAN_POINT('Origin',(-0.04655,-0.0222,0.053125));
#5946=CARTESIAN_POINT('Origin',(-0.04655,-0.0222,0.043125));
#5947=CARTESIAN_POINT('Origin',(-0.06655,-0.009975,0.02565));
#5948=CARTESIAN_POINT('Origin',(-0.06655,-0.009975,0.02565));
#5949=CARTESIAN_POINT('Origin',(-0.06855,-0.009975,0.02565));
#5950=CARTESIAN_POINT('',(-0.06855,-0.0222,0.003175));
#5951=CARTESIAN_POINT('Origin',(-0.06855,-0.0222,-0.001825));
#5952=CARTESIAN_POINT('',(-0.06855,-0.0272,0.008175));
#5953=CARTESIAN_POINT('Origin',(-0.06855,-0.0222,0.008175));
#5954=CARTESIAN_POINT('',(-0.06855,-0.0272,0.043125));
#5955=CARTESIAN_POINT('',(-0.06855,-0.0272,0.02565));
#5956=CARTESIAN_POINT('',(-0.06855,-0.0222,0.048125));
#5957=CARTESIAN_POINT('Origin',(-0.06855,-0.0222,0.043125));
#5958=CARTESIAN_POINT('Origin',(-0.06855,-0.0222,0.053125));
#5959=CARTESIAN_POINT('Origin',(-0.06855,-0.0122,0.061125));
#5960=CARTESIAN_POINT('Origin',(-0.06855,-0.00775,0.061125));
#5961=CARTESIAN_POINT('Origin',(-0.06855,-0.00775,-0.009825));
#5962=CARTESIAN_POINT('Origin',(-0.06855,-0.0122,-0.009825));
#5963=CARTESIAN_POINT('Origin',(-0.06655,-0.0122,0.061125));
#5964=CARTESIAN_POINT('Origin',(-0.06655,-0.00775,0.061125));
#5965=CARTESIAN_POINT('Origin',(-0.06655,-0.00775,-0.009825));
#5966=CARTESIAN_POINT('Origin',(-0.06655,-0.0122,-0.009825));
#5967=CARTESIAN_POINT('Origin',(-0.05755,-0.0272,0.02565));
#5968=CARTESIAN_POINT('',(-0.0622553825561797,-0.0272,0.008175));
#5969=CARTESIAN_POINT('',(-0.04655,-0.0272,0.008175));
#5970=CARTESIAN_POINT('',(-0.05755,-0.0272,0.0218));
#5971=CARTESIAN_POINT('Origin',(-0.05755,-0.0272,0.014175));
#5972=CARTESIAN_POINT('',(-0.0528446174438203,-0.0272,0.008175));
#5973=CARTESIAN_POINT('Origin',(-0.05755,-0.0272,0.014175));
#5974=CARTESIAN_POINT('',(-0.04655,-0.0272,0.008175));
#5975=CARTESIAN_POINT('',(-0.0528446174438203,-0.0272,0.043125));
#5976=CARTESIAN_POINT('',(-0.05755,-0.0272,0.043125));
#5977=CARTESIAN_POINT('',(-0.0622553825561797,-0.0272,0.043125));
#5978=CARTESIAN_POINT('Origin',(-0.05755,-0.0272,0.037125));
#5979=CARTESIAN_POINT('',(-0.05755,-0.0272,0.043125));
#5980=CARTESIAN_POINT('Origin',(-0.05755,-0.0022,0.037125));
#5981=CARTESIAN_POINT('',(-0.05755,-0.0269285700798444,0.04475));
#5982=CARTESIAN_POINT('',(-0.05755,-0.0022,0.04475));
#5983=CARTESIAN_POINT('Ctrl Pts',(-0.0622553825561797,-0.0272,0.043125));
#5984=CARTESIAN_POINT('Ctrl Pts',(-0.0617185912965407,-0.0272,0.0435459680382359));
#5985=CARTESIAN_POINT('Ctrl Pts',(-0.0611100942808263,-0.027146490983882,
0.0439040351600042));
#5986=CARTESIAN_POINT('Ctrl Pts',(-0.0595292759370733,-0.0270066019492738,
0.0445577665669935));
#5987=CARTESIAN_POINT('Ctrl Pts',(-0.058511387005684,-0.0269285700798444,
0.04475));
#5988=CARTESIAN_POINT('Ctrl Pts',(-0.05755,-0.0269285700798444,0.04475));
#5989=CARTESIAN_POINT('Ctrl Pts',(-0.05755,-0.0269285700798444,0.04475));
#5990=CARTESIAN_POINT('Ctrl Pts',(-0.056588612994316,-0.0269285700798444,
0.04475));
#5991=CARTESIAN_POINT('Ctrl Pts',(-0.0555707240629267,-0.0270066019492738,
0.0445577665669935));
#5992=CARTESIAN_POINT('Ctrl Pts',(-0.0539899057191737,-0.027146490983882,
0.0439040351600042));
#5993=CARTESIAN_POINT('Ctrl Pts',(-0.0533814087034593,-0.0272,0.0435459680382359));
#5994=CARTESIAN_POINT('Ctrl Pts',(-0.0528446174438203,-0.0272,0.043125));
#5995=CARTESIAN_POINT('Origin',(-0.05755,-0.0022,0.014175));
#5996=CARTESIAN_POINT('',(-0.05755,-0.0022,0.0218));
#5997=CARTESIAN_POINT('Ctrl Pts',(-0.0622553825561797,-0.0272,0.00817500000000001));
#5998=CARTESIAN_POINT('Ctrl Pts',(-0.0617185912965407,-0.0272,0.00775403196176415));
#5999=CARTESIAN_POINT('Ctrl Pts',(-0.0611100942808263,-0.027146490983882,
0.00739596483999584));
#6000=CARTESIAN_POINT('Ctrl Pts',(-0.0595292759370733,-0.0270066019492738,
0.00674223343300649));
#6001=CARTESIAN_POINT('Ctrl Pts',(-0.058511387005684,-0.0269285700798444,
0.00655));
#6002=CARTESIAN_POINT('Ctrl Pts',(-0.056588612994316,-0.0269285700798444,
0.00655));
#6003=CARTESIAN_POINT('Ctrl Pts',(-0.0555707240629267,-0.0270066019492738,
0.00674223343300649));
#6004=CARTESIAN_POINT('Ctrl Pts',(-0.0539899057191737,-0.027146490983882,
0.00739596483999584));
#6005=CARTESIAN_POINT('Ctrl Pts',(-0.0533814087034593,-0.0272,0.00775403196176415));
#6006=CARTESIAN_POINT('Ctrl Pts',(-0.0528446174438203,-0.0272,0.00817500000000001));
#6007=CARTESIAN_POINT('Origin',(-0.05755,-0.0222,0.008175));
#6008=CARTESIAN_POINT('',(-0.06855,-0.0222,0.003175));
#6009=CARTESIAN_POINT('Origin',(-0.05755,-0.0222,-0.001825));
#6010=CARTESIAN_POINT('Origin',(-0.05755,-0.0222,0.043125));
#6011=CARTESIAN_POINT('',(-0.05755,-0.0222,0.048125));
#6012=CARTESIAN_POINT('Origin',(-0.06655,-0.0222,0.053125));
#6306=UNCERTAINTY_MEASURE_WITH_UNIT(LENGTH_MEASURE(1.E-5),#6349,
'DISTANCE_ACCURACY_VALUE',
'Maximum model space distance between geometric entities at asserted c
onnectivities');
#6323=UNCERTAINTY_MEASURE_WITH_UNIT(LENGTH_MEASURE(1.E-5),#6349,
'DISTANCE_ACCURACY_VALUE',
'Maximum model space distance between geometric entities at asserted c
onnectivities');
#6331=(
GEOMETRIC_REPRESENTATION_CONTEXT(3)
GLOBAL_UNCERTAINTY_ASSIGNED_CONTEXT((#6306))
GLOBAL_UNIT_ASSIGNED_CONTEXT((#6349,#6350,#6351))
REPRESENTATION_CONTEXT('','3D')
);
#6348=(
GEOMETRIC_REPRESENTATION_CONTEXT(3)
GLOBAL_UNCERTAINTY_ASSIGNED_CONTEXT((#6323))
GLOBAL_UNIT_ASSIGNED_CONTEXT((#6349,#6350,#6351))
REPRESENTATION_CONTEXT('','3D')
);
#6349=(
LENGTH_UNIT()
NAMED_UNIT(*)
SI_UNIT($,.METRE.)
);
#6350=(
NAMED_UNIT(*)
PLANE_ANGLE_UNIT()
SI_UNIT($,.RADIAN.)
);
#6351=(
NAMED_UNIT(*)
SI_UNIT($,.STERADIAN.)
SOLID_ANGLE_UNIT()
);
#6359=SHAPE_DEFINITION_REPRESENTATION(#6383,#6483);
#6383=PRODUCT_DEFINITION_SHAPE('',$,#6508);
#6483=SHAPE_REPRESENTATION('',(#3731),#6331);
#6500=PRODUCT_DEFINITION_CONTEXT('part definition',#6574,'design');
#6508=PRODUCT_DEFINITION('End Cap Left','End Cap Left',#6532,#6500);
#6532=PRODUCT_DEFINITION_FORMATION('',$,#6583);
#6574=APPLICATION_CONTEXT('Managed model based 3d engineering');
#6575=PRODUCT_CONTEXT('part definition',#6574,'mechanical');
#6583=PRODUCT('End Cap Left','End Cap Left',
'LEGAL AND USAGE DISCLAIMER: this Data/Model is provided \X2\201C\X0\A
S IS\X2\201D\X0\ for informational and representational only. It is a 
geometric approximation and is NOT engineered, certified, or guarantee
d for dimensional accuracy, exact tolerances, or production-level prec
ision. Vendor disclaims all implied warranties including fitness for a
 particular purpose. DO NOT USE FOR DIRECT PHYSICAL MANUFACTURING, AUT
OMATED PRODUCTION, OR SAFETY-CRITICAL SYSTEMS without independent engi
neering verification and resolution of any design discrepancies.',(#6575));
#6604=PRESENTATION_STYLE_ASSIGNMENT((#6610));
#6610=SURFACE_STYLE_USAGE(.BOTH.,#6616);
#6616=SURFACE_SIDE_STYLE('',(#6622));
#6622=SURFACE_STYLE_FILL_AREA(#6628);
#6628=FILL_AREA_STYLE('Opaque(25,25,25)',(#6634));
#6634=FILL_AREA_STYLE_COLOUR('Opaque(25,25,25)',#6640);
#6640=COLOUR_RGB('Opaque(25,25,25)',0.0980392156862745,0.0980392156862745,
0.0980392156862745);
ENDSEC;
END-ISO-10303-21;
